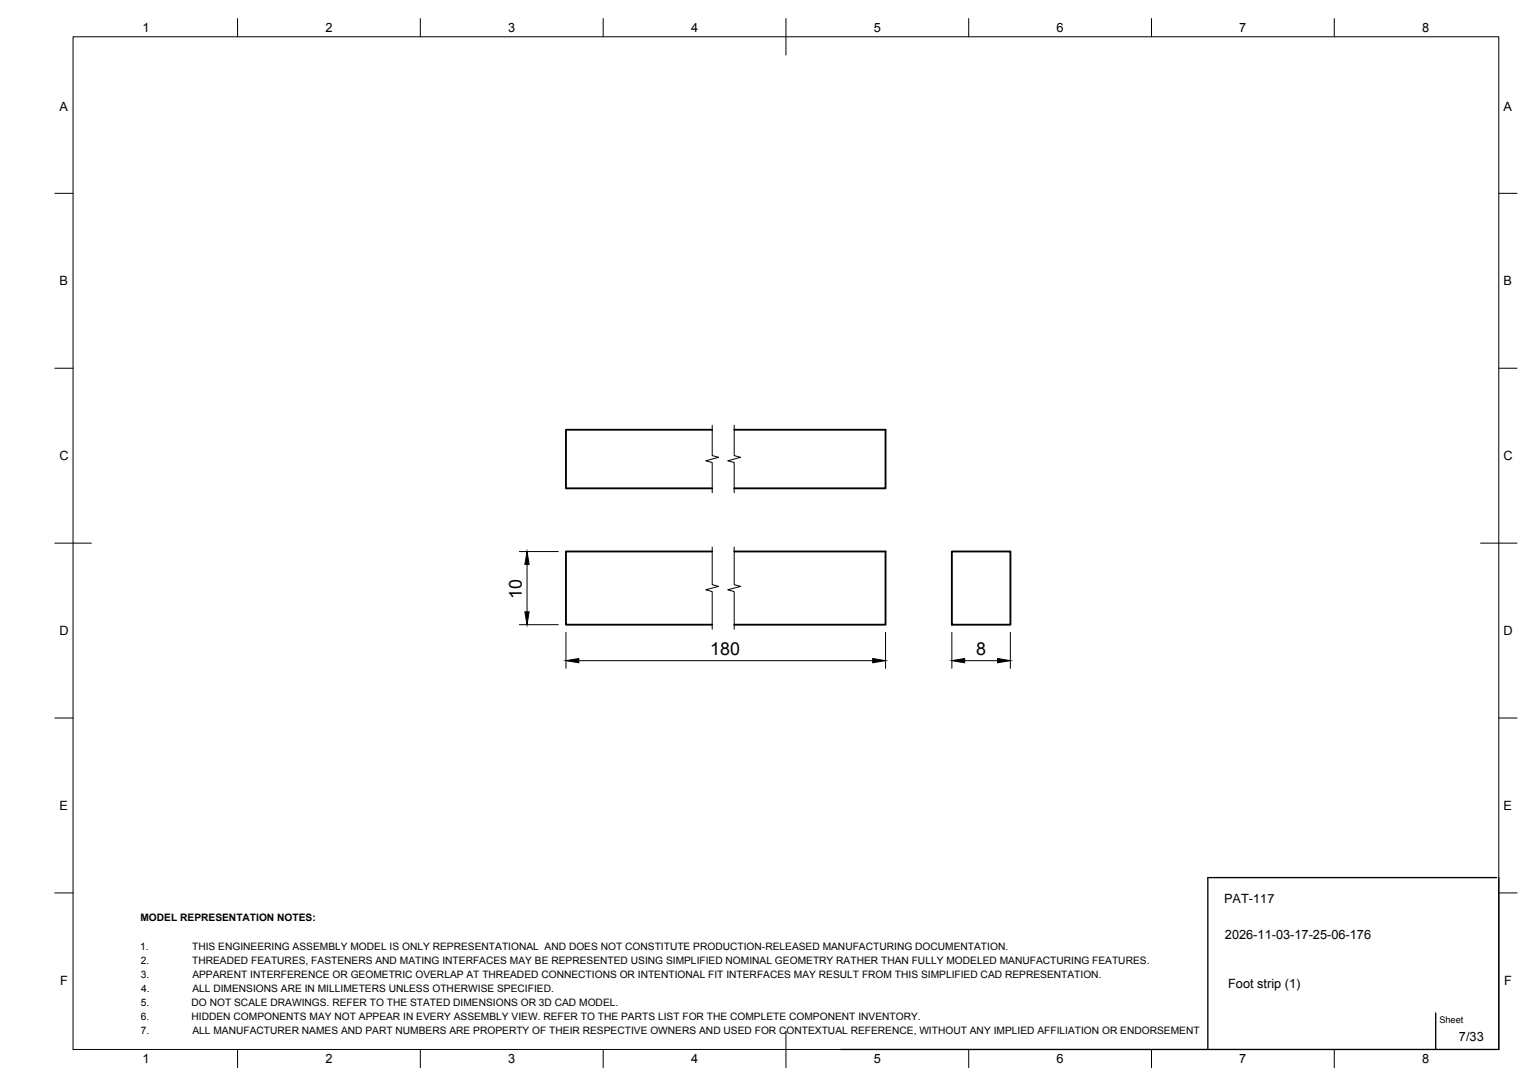
ISO-10303-21;
HEADER;
/* Generated by software containing ST-Developer
 * from STEP Tools, Inc. (www.steptools.com) 
 */

FILE_DESCRIPTION(
/* description */ ('Counterbalanced vertical column'),
/* implementation_level */ '2;1');

FILE_NAME(
/* name */ 'Foot strip (1).step',
/* time_stamp */ '2026-10-29T16:47:22-07:00',
/* author */ (''),
/* organization */ (''),
/* preprocessor_version */ 'ST-DEVELOPER v20.2',
/* originating_system */ 'Autodesk Translation Framework v15.17.0.0',
/* authorisation */ '');

FILE_SCHEMA (('AUTOMOTIVE_DESIGN { 1 0 10303 214 3 1 1 }'));
ENDSEC;

DATA;
#10=MECHANICAL_DESIGN_GEOMETRIC_PRESENTATION_REPRESENTATION('',(#352),#15040);
#282=SHAPE_REPRESENTATION_RELATIONSHIP('SRR','None',#15186,#317);
#317=ADVANCED_BREP_SHAPE_REPRESENTATION('',(#387),#15005);
#352=STYLED_ITEM('',(#15443),#387);
#387=MANIFOLD_SOLID_BREP('Body1',#7075);
#547=PLANE('',#7534);
#548=PLANE('',#7535);
#549=PLANE('',#7536);
#550=PLANE('',#7537);
#551=PLANE('',#7538);
#552=PLANE('',#7539);
#847=FACE_OUTER_BOUND('',#1258,.T.);
#848=FACE_OUTER_BOUND('',#1259,.T.);
#849=FACE_OUTER_BOUND('',#1260,.T.);
#850=FACE_OUTER_BOUND('',#1261,.T.);
#851=FACE_OUTER_BOUND('',#1262,.T.);
#852=FACE_OUTER_BOUND('',#1263,.T.);
#1258=EDGE_LOOP('',(#4866,#4867,#4868,#4869));
#1259=EDGE_LOOP('',(#4870,#4871,#4872,#4873));
#1260=EDGE_LOOP('',(#4874,#4875,#4876,#4877));
#1261=EDGE_LOOP('',(#4878,#4879,#4880,#4881));
#1262=EDGE_LOOP('',(#4882,#4883,#4884,#4885));
#1263=EDGE_LOOP('',(#4886,#4887,#4888,#4889));
#1780=LINE('',#10432,#2451);
#1781=LINE('',#10434,#2452);
#1782=LINE('',#10436,#2453);
#1783=LINE('',#10437,#2454);
#1784=LINE('',#10440,#2455);
#1785=LINE('',#10442,#2456);
#1786=LINE('',#10443,#2457);
#1787=LINE('',#10446,#2458);
#1788=LINE('',#10448,#2459);
#1789=LINE('',#10449,#2460);
#1790=LINE('',#10451,#2461);
#1791=LINE('',#10452,#2462);
#2451=VECTOR('',#8324,1.);
#2452=VECTOR('',#8325,1.);
#2453=VECTOR('',#8326,1.);
#2454=VECTOR('',#8327,1.);
#2455=VECTOR('',#8330,1.);
#2456=VECTOR('',#8331,1.);
#2457=VECTOR('',#8332,1.);
#2458=VECTOR('',#8335,1.);
#2459=VECTOR('',#8336,1.);
#2460=VECTOR('',#8337,1.);
#2461=VECTOR('',#8340,1.);
#2462=VECTOR('',#8341,1.);
#3332=VERTEX_POINT('',#10430);
#3333=VERTEX_POINT('',#10431);
#3334=VERTEX_POINT('',#10433);
#3335=VERTEX_POINT('',#10435);
#3336=VERTEX_POINT('',#10439);
#3337=VERTEX_POINT('',#10441);
#3338=VERTEX_POINT('',#10445);
#3339=VERTEX_POINT('',#10447);
#3934=EDGE_CURVE('',#3332,#3333,#1780,.T.);
#3935=EDGE_CURVE('',#3333,#3334,#1781,.T.);
#3936=EDGE_CURVE('',#3335,#3334,#1782,.T.);
#3937=EDGE_CURVE('',#3332,#3335,#1783,.T.);
#3938=EDGE_CURVE('',#3336,#3332,#1784,.T.);
#3939=EDGE_CURVE('',#3337,#3335,#1785,.T.);
#3940=EDGE_CURVE('',#3336,#3337,#1786,.T.);
#3941=EDGE_CURVE('',#3338,#3336,#1787,.T.);
#3942=EDGE_CURVE('',#3339,#3337,#1788,.T.);
#3943=EDGE_CURVE('',#3338,#3339,#1789,.T.);
#3944=EDGE_CURVE('',#3333,#3338,#1790,.T.);
#3945=EDGE_CURVE('',#3334,#3339,#1791,.T.);
#4866=ORIENTED_EDGE('',*,*,#3934,.T.);
#4867=ORIENTED_EDGE('',*,*,#3935,.T.);
#4868=ORIENTED_EDGE('',*,*,#3936,.F.);
#4869=ORIENTED_EDGE('',*,*,#3937,.F.);
#4870=ORIENTED_EDGE('',*,*,#3938,.T.);
#4871=ORIENTED_EDGE('',*,*,#3937,.T.);
#4872=ORIENTED_EDGE('',*,*,#3939,.F.);
#4873=ORIENTED_EDGE('',*,*,#3940,.F.);
#4874=ORIENTED_EDGE('',*,*,#3941,.T.);
#4875=ORIENTED_EDGE('',*,*,#3940,.T.);
#4876=ORIENTED_EDGE('',*,*,#3942,.F.);
#4877=ORIENTED_EDGE('',*,*,#3943,.F.);
#4878=ORIENTED_EDGE('',*,*,#3944,.T.);
#4879=ORIENTED_EDGE('',*,*,#3943,.T.);
#4880=ORIENTED_EDGE('',*,*,#3945,.F.);
#4881=ORIENTED_EDGE('',*,*,#3935,.F.);
#4882=ORIENTED_EDGE('',*,*,#3945,.T.);
#4883=ORIENTED_EDGE('',*,*,#3942,.T.);
#4884=ORIENTED_EDGE('',*,*,#3939,.T.);
#4885=ORIENTED_EDGE('',*,*,#3936,.T.);
#4886=ORIENTED_EDGE('',*,*,#3944,.F.);
#4887=ORIENTED_EDGE('',*,*,#3934,.F.);
#4888=ORIENTED_EDGE('',*,*,#3938,.F.);
#4889=ORIENTED_EDGE('',*,*,#3941,.F.);
#6689=ADVANCED_FACE('',(#847),#547,.T.);
#6690=ADVANCED_FACE('',(#848),#548,.T.);
#6691=ADVANCED_FACE('',(#849),#549,.T.);
#6692=ADVANCED_FACE('',(#850),#550,.T.);
#6693=ADVANCED_FACE('',(#851),#551,.T.);
#6694=ADVANCED_FACE('',(#852),#552,.F.);
#7075=CLOSED_SHELL('',(#6689,#6690,#6691,#6692,#6693,#6694));
#7533=AXIS2_PLACEMENT_3D('',#10428,#8320,#8321);
#7534=AXIS2_PLACEMENT_3D('',#10429,#8322,#8323);
#7535=AXIS2_PLACEMENT_3D('',#10438,#8328,#8329);
#7536=AXIS2_PLACEMENT_3D('',#10444,#8333,#8334);
#7537=AXIS2_PLACEMENT_3D('',#10450,#8338,#8339);
#7538=AXIS2_PLACEMENT_3D('',#10453,#8342,#8343);
#7539=AXIS2_PLACEMENT_3D('',#10454,#8344,#8345);
#8320=DIRECTION('axis',(0.,0.,1.));
#8321=DIRECTION('refdir',(1.,0.,0.));
#8322=DIRECTION('center_axis',(0.,1.,0.));
#8323=DIRECTION('ref_axis',(-1.,0.,0.));
#8324=DIRECTION('',(-1.,0.,0.));
#8325=DIRECTION('',(0.,0.,1.));
#8326=DIRECTION('',(-1.,0.,0.));
#8327=DIRECTION('',(0.,0.,1.));
#8328=DIRECTION('center_axis',(1.,0.,0.));
#8329=DIRECTION('ref_axis',(0.,1.,0.));
#8330=DIRECTION('',(0.,1.,0.));
#8331=DIRECTION('',(0.,1.,0.));
#8332=DIRECTION('',(0.,0.,1.));
#8333=DIRECTION('center_axis',(0.,-1.,0.));
#8334=DIRECTION('ref_axis',(1.,0.,0.));
#8335=DIRECTION('',(1.,0.,0.));
#8336=DIRECTION('',(1.,0.,0.));
#8337=DIRECTION('',(0.,0.,1.));
#8338=DIRECTION('center_axis',(-1.,0.,0.));
#8339=DIRECTION('ref_axis',(0.,-1.,0.));
#8340=DIRECTION('',(0.,-1.,0.));
#8341=DIRECTION('',(0.,-1.,0.));
#8342=DIRECTION('center_axis',(0.,0.,1.));
#8343=DIRECTION('ref_axis',(1.,0.,0.));
#8344=DIRECTION('center_axis',(0.,0.,1.));
#8345=DIRECTION('ref_axis',(1.,0.,0.));
#10428=CARTESIAN_POINT('',(0.,0.,0.));
#10429=CARTESIAN_POINT('Origin',(6.,6.,-1.8));
#10430=CARTESIAN_POINT('',(6.,6.,-1.8));
#10431=CARTESIAN_POINT('',(-12.,6.,-1.8));
#10432=CARTESIAN_POINT('',(6.,6.,-1.8));
#10433=CARTESIAN_POINT('',(-12.,6.,-1.));
#10434=CARTESIAN_POINT('',(-12.,6.,-1.8));
#10435=CARTESIAN_POINT('',(6.,6.,-1.));
#10436=CARTESIAN_POINT('',(6.,6.,-1.));
#10437=CARTESIAN_POINT('',(6.,6.,-1.8));
#10438=CARTESIAN_POINT('Origin',(6.,5.,-1.8));
#10439=CARTESIAN_POINT('',(6.,5.,-1.8));
#10440=CARTESIAN_POINT('',(6.,5.,-1.8));
#10441=CARTESIAN_POINT('',(6.,5.,-1.));
#10442=CARTESIAN_POINT('',(6.,5.,-1.));
#10443=CARTESIAN_POINT('',(6.,5.,-1.8));
#10444=CARTESIAN_POINT('Origin',(-12.,5.,-1.8));
#10445=CARTESIAN_POINT('',(-12.,5.,-1.8));
#10446=CARTESIAN_POINT('',(-12.,5.,-1.8));
#10447=CARTESIAN_POINT('',(-12.,5.,-1.));
#10448=CARTESIAN_POINT('',(-12.,5.,-1.));
#10449=CARTESIAN_POINT('',(-12.,5.,-1.8));
#10450=CARTESIAN_POINT('Origin',(-12.,6.,-1.8));
#10451=CARTESIAN_POINT('',(-12.,6.,-1.8));
#10452=CARTESIAN_POINT('',(-12.,6.,-1.));
#10453=CARTESIAN_POINT('Origin',(-3.,5.5,-1.));
#10454=CARTESIAN_POINT('Origin',(-3.,5.5,-1.8));
#14965=UNCERTAINTY_MEASURE_WITH_UNIT(LENGTH_MEASURE(0.001),#15041,
'DISTANCE_ACCURACY_VALUE',
'Maximum model space distance between geometric entities at asserted c
onnectivities');
#15000=UNCERTAINTY_MEASURE_WITH_UNIT(LENGTH_MEASURE(0.001),#15041,
'DISTANCE_ACCURACY_VALUE',
'Maximum model space distance between geometric entities at asserted c
onnectivities');
#15005=(
GEOMETRIC_REPRESENTATION_CONTEXT(3)
GLOBAL_UNCERTAINTY_ASSIGNED_CONTEXT((#14965))
GLOBAL_UNIT_ASSIGNED_CONTEXT((#15041,#15043,#15044))
REPRESENTATION_CONTEXT('','3D')
);
#15040=(
GEOMETRIC_REPRESENTATION_CONTEXT(3)
GLOBAL_UNCERTAINTY_ASSIGNED_CONTEXT((#15000))
GLOBAL_UNIT_ASSIGNED_CONTEXT((#15041,#15043,#15044))
REPRESENTATION_CONTEXT('','3D')
);
#15041=(
LENGTH_UNIT()
NAMED_UNIT(*)
SI_UNIT(.CENTI.,.METRE.)
);
#15043=(
NAMED_UNIT(*)
PLANE_ANGLE_UNIT()
SI_UNIT($,.RADIAN.)
);
#15044=(
NAMED_UNIT(*)
SI_UNIT($,.STERADIAN.)
SOLID_ANGLE_UNIT()
);
#15049=SHAPE_DEFINITION_REPRESENTATION(#15088,#15186);
#15088=PRODUCT_DEFINITION_SHAPE('',$,#15226);
#15186=SHAPE_REPRESENTATION('',(#7533),#15005);
#15221=PRODUCT_DEFINITION_CONTEXT('part definition',#15340,'design');
#15226=PRODUCT_DEFINITION('Foot strip (1)','Foot strip (1)',#15265,#15221);
#15265=PRODUCT_DEFINITION_FORMATION('',$,#15346);
#15340=APPLICATION_CONTEXT(
'Core Data for Automotive Mechanical Design Process');
#15341=PRODUCT_CONTEXT('part definition',#15340,'mechanical');
#15346=PRODUCT('Foot strip (1)','Foot strip (1)','Foot strip (1)',(#15341));
#15437=COLOUR_RGB('Light Blue',0.38,0.62,0.78);
#15438=FILL_AREA_STYLE_COLOUR('',#15437);
#15439=FILL_AREA_STYLE('',(#15438));
#15440=SURFACE_STYLE_FILL_AREA(#15439);
#15441=SURFACE_SIDE_STYLE('',(#15440));
#15442=SURFACE_STYLE_USAGE(.BOTH.,#15441);
#15443=PRESENTATION_STYLE_ASSIGNMENT((#15442));
ENDSEC;
END-ISO-10303-21;
